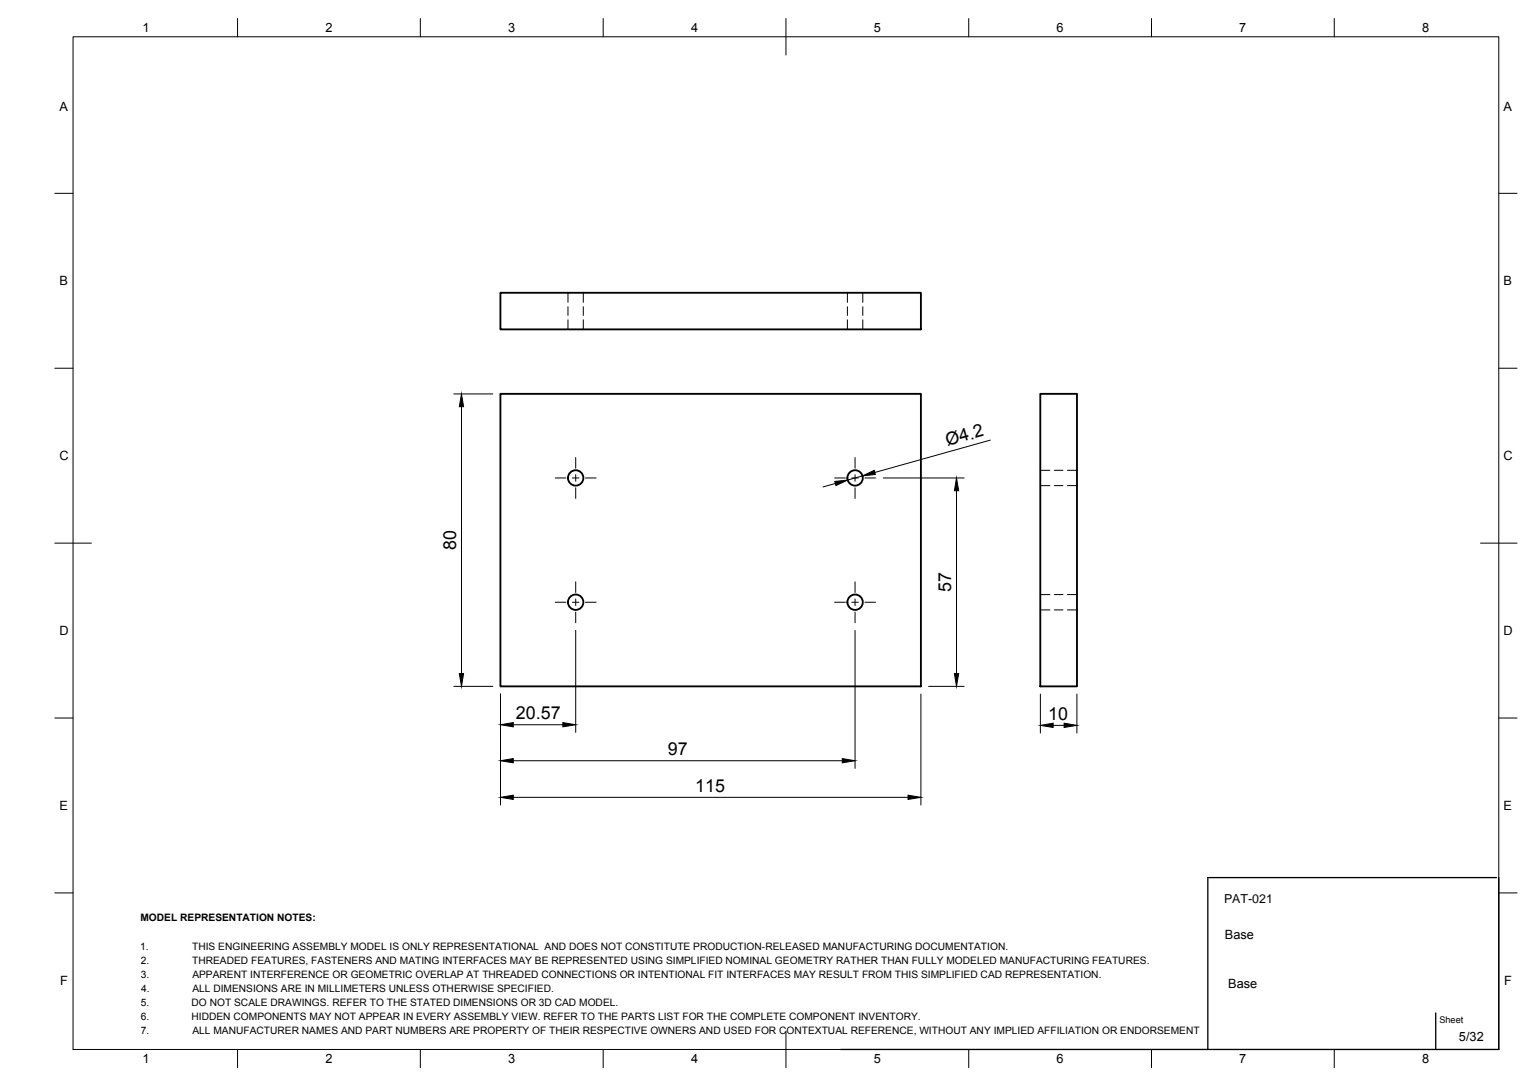
ISO-10303-21;
HEADER;
/* Generated by software containing ST-Developer
 * from STEP Tools, Inc. (www.steptools.com) 
 */

FILE_DESCRIPTION(
/* description */ ('Chain-less indexing wheel (Geneva) drive'),
/* implementation_level */ '2;1');

FILE_NAME(
/* name */ 'Base.step',
/* time_stamp */ '2026-10-28T03:25:22-07:00',
/* author */ (''),
/* organization */ (''),
/* preprocessor_version */ 'ST-DEVELOPER v20.2',
/* originating_system */ 'Autodesk Translation Framework v15.17.0.0',
/* authorisation */ '');

FILE_SCHEMA (('AUTOMOTIVE_DESIGN { 1 0 10303 214 3 1 1 }'));
ENDSEC;

DATA;
#10=MECHANICAL_DESIGN_GEOMETRIC_PRESENTATION_REPRESENTATION('',(#303),#10957);
#253=SHAPE_REPRESENTATION_RELATIONSHIP('SRR','None',#11066,#278);
#278=ADVANCED_BREP_SHAPE_REPRESENTATION('',(#336),#10929);
#303=STYLED_ITEM('',(#11266),#336);
#336=MANIFOLD_SOLID_BREP('Body1',#5699);
#367=FACE_BOUND('',#994,.T.);
#368=FACE_BOUND('',#995,.T.);
#369=FACE_BOUND('',#996,.T.);
#370=FACE_BOUND('',#997,.T.);
#371=FACE_BOUND('',#999,.T.);
#372=FACE_BOUND('',#1000,.T.);
#373=FACE_BOUND('',#1001,.T.);
#374=FACE_BOUND('',#1002,.T.);
#472=PLANE('',#6025);
#473=PLANE('',#6026);
#474=PLANE('',#6027);
#475=PLANE('',#6028);
#476=PLANE('',#6029);
#477=PLANE('',#6030);
#652=FACE_OUTER_BOUND('',#985,.T.);
#653=FACE_OUTER_BOUND('',#986,.T.);
#654=FACE_OUTER_BOUND('',#987,.T.);
#655=FACE_OUTER_BOUND('',#988,.T.);
#656=FACE_OUTER_BOUND('',#989,.T.);
#657=FACE_OUTER_BOUND('',#990,.T.);
#658=FACE_OUTER_BOUND('',#991,.T.);
#659=FACE_OUTER_BOUND('',#992,.T.);
#660=FACE_OUTER_BOUND('',#993,.T.);
#661=FACE_OUTER_BOUND('',#998,.T.);
#985=EDGE_LOOP('',(#3747,#3748,#3749,#3750));
#986=EDGE_LOOP('',(#3751,#3752,#3753,#3754));
#987=EDGE_LOOP('',(#3755,#3756,#3757,#3758));
#988=EDGE_LOOP('',(#3759,#3760,#3761,#3762));
#989=EDGE_LOOP('',(#3763,#3764,#3765,#3766));
#990=EDGE_LOOP('',(#3767,#3768,#3769,#3770));
#991=EDGE_LOOP('',(#3771,#3772,#3773,#3774));
#992=EDGE_LOOP('',(#3775,#3776,#3777,#3778));
#993=EDGE_LOOP('',(#3779,#3780,#3781,#3782));
#994=EDGE_LOOP('',(#3783));
#995=EDGE_LOOP('',(#3784));
#996=EDGE_LOOP('',(#3785));
#997=EDGE_LOOP('',(#3786));
#998=EDGE_LOOP('',(#3787,#3788,#3789,#3790));
#999=EDGE_LOOP('',(#3791));
#1000=EDGE_LOOP('',(#3792));
#1001=EDGE_LOOP('',(#3793));
#1002=EDGE_LOOP('',(#3794));
#1423=LINE('',#8608,#1797);
#1424=LINE('',#8614,#1798);
#1425=LINE('',#8620,#1799);
#1426=LINE('',#8626,#1800);
#1427=LINE('',#8631,#1801);
#1428=LINE('',#8633,#1802);
#1429=LINE('',#8635,#1803);
#1430=LINE('',#8636,#1804);
#1431=LINE('',#8639,#1805);
#1432=LINE('',#8641,#1806);
#1433=LINE('',#8642,#1807);
#1434=LINE('',#8645,#1808);
#1435=LINE('',#8647,#1809);
#1436=LINE('',#8648,#1810);
#1437=LINE('',#8650,#1811);
#1438=LINE('',#8651,#1812);
#1797=VECTOR('',#6759,0.21);
#1798=VECTOR('',#6766,0.21);
#1799=VECTOR('',#6773,0.21);
#1800=VECTOR('',#6780,0.21);
#1801=VECTOR('',#6785,1.);
#1802=VECTOR('',#6786,1.);
#1803=VECTOR('',#6787,1.);
#1804=VECTOR('',#6788,1.);
#1805=VECTOR('',#6791,1.);
#1806=VECTOR('',#6792,1.);
#1807=VECTOR('',#6793,1.);
#1808=VECTOR('',#6796,1.);
#1809=VECTOR('',#6797,1.);
#1810=VECTOR('',#6798,1.);
#1811=VECTOR('',#6801,1.);
#1812=VECTOR('',#6802,1.);
#2171=CIRCLE('',#6014,0.21);
#2172=CIRCLE('',#6015,0.21);
#2173=CIRCLE('',#6017,0.21);
#2174=CIRCLE('',#6018,0.21);
#2175=CIRCLE('',#6020,0.21);
#2176=CIRCLE('',#6021,0.21);
#2177=CIRCLE('',#6023,0.21);
#2178=CIRCLE('',#6024,0.21);
#2505=VERTEX_POINT('',#8605);
#2506=VERTEX_POINT('',#8607);
#2507=VERTEX_POINT('',#8611);
#2508=VERTEX_POINT('',#8613);
#2509=VERTEX_POINT('',#8617);
#2510=VERTEX_POINT('',#8619);
#2511=VERTEX_POINT('',#8623);
#2512=VERTEX_POINT('',#8625);
#2513=VERTEX_POINT('',#8629);
#2514=VERTEX_POINT('',#8630);
#2515=VERTEX_POINT('',#8632);
#2516=VERTEX_POINT('',#8634);
#2517=VERTEX_POINT('',#8638);
#2518=VERTEX_POINT('',#8640);
#2519=VERTEX_POINT('',#8644);
#2520=VERTEX_POINT('',#8646);
#2999=EDGE_CURVE('',#2505,#2505,#2171,.T.);
#3000=EDGE_CURVE('',#2505,#2506,#1423,.T.);
#3001=EDGE_CURVE('',#2506,#2506,#2172,.T.);
#3002=EDGE_CURVE('',#2507,#2507,#2173,.T.);
#3003=EDGE_CURVE('',#2507,#2508,#1424,.T.);
#3004=EDGE_CURVE('',#2508,#2508,#2174,.T.);
#3005=EDGE_CURVE('',#2509,#2509,#2175,.T.);
#3006=EDGE_CURVE('',#2509,#2510,#1425,.T.);
#3007=EDGE_CURVE('',#2510,#2510,#2176,.T.);
#3008=EDGE_CURVE('',#2511,#2511,#2177,.T.);
#3009=EDGE_CURVE('',#2511,#2512,#1426,.T.);
#3010=EDGE_CURVE('',#2512,#2512,#2178,.T.);
#3011=EDGE_CURVE('',#2513,#2514,#1427,.T.);
#3012=EDGE_CURVE('',#2514,#2515,#1428,.T.);
#3013=EDGE_CURVE('',#2516,#2515,#1429,.T.);
#3014=EDGE_CURVE('',#2513,#2516,#1430,.T.);
#3015=EDGE_CURVE('',#2517,#2513,#1431,.T.);
#3016=EDGE_CURVE('',#2518,#2516,#1432,.T.);
#3017=EDGE_CURVE('',#2517,#2518,#1433,.T.);
#3018=EDGE_CURVE('',#2519,#2517,#1434,.T.);
#3019=EDGE_CURVE('',#2520,#2518,#1435,.T.);
#3020=EDGE_CURVE('',#2519,#2520,#1436,.T.);
#3021=EDGE_CURVE('',#2514,#2519,#1437,.T.);
#3022=EDGE_CURVE('',#2515,#2520,#1438,.T.);
#3747=ORIENTED_EDGE('',*,*,#2999,.F.);
#3748=ORIENTED_EDGE('',*,*,#3000,.T.);
#3749=ORIENTED_EDGE('',*,*,#3001,.F.);
#3750=ORIENTED_EDGE('',*,*,#3000,.F.);
#3751=ORIENTED_EDGE('',*,*,#3002,.F.);
#3752=ORIENTED_EDGE('',*,*,#3003,.T.);
#3753=ORIENTED_EDGE('',*,*,#3004,.F.);
#3754=ORIENTED_EDGE('',*,*,#3003,.F.);
#3755=ORIENTED_EDGE('',*,*,#3005,.F.);
#3756=ORIENTED_EDGE('',*,*,#3006,.T.);
#3757=ORIENTED_EDGE('',*,*,#3007,.F.);
#3758=ORIENTED_EDGE('',*,*,#3006,.F.);
#3759=ORIENTED_EDGE('',*,*,#3008,.F.);
#3760=ORIENTED_EDGE('',*,*,#3009,.T.);
#3761=ORIENTED_EDGE('',*,*,#3010,.F.);
#3762=ORIENTED_EDGE('',*,*,#3009,.F.);
#3763=ORIENTED_EDGE('',*,*,#3011,.T.);
#3764=ORIENTED_EDGE('',*,*,#3012,.T.);
#3765=ORIENTED_EDGE('',*,*,#3013,.F.);
#3766=ORIENTED_EDGE('',*,*,#3014,.F.);
#3767=ORIENTED_EDGE('',*,*,#3015,.T.);
#3768=ORIENTED_EDGE('',*,*,#3014,.T.);
#3769=ORIENTED_EDGE('',*,*,#3016,.F.);
#3770=ORIENTED_EDGE('',*,*,#3017,.F.);
#3771=ORIENTED_EDGE('',*,*,#3018,.T.);
#3772=ORIENTED_EDGE('',*,*,#3017,.T.);
#3773=ORIENTED_EDGE('',*,*,#3019,.F.);
#3774=ORIENTED_EDGE('',*,*,#3020,.F.);
#3775=ORIENTED_EDGE('',*,*,#3021,.T.);
#3776=ORIENTED_EDGE('',*,*,#3020,.T.);
#3777=ORIENTED_EDGE('',*,*,#3022,.F.);
#3778=ORIENTED_EDGE('',*,*,#3012,.F.);
#3779=ORIENTED_EDGE('',*,*,#3022,.T.);
#3780=ORIENTED_EDGE('',*,*,#3019,.T.);
#3781=ORIENTED_EDGE('',*,*,#3016,.T.);
#3782=ORIENTED_EDGE('',*,*,#3013,.T.);
#3783=ORIENTED_EDGE('',*,*,#3001,.T.);
#3784=ORIENTED_EDGE('',*,*,#3004,.T.);
#3785=ORIENTED_EDGE('',*,*,#3007,.T.);
#3786=ORIENTED_EDGE('',*,*,#3010,.T.);
#3787=ORIENTED_EDGE('',*,*,#3021,.F.);
#3788=ORIENTED_EDGE('',*,*,#3011,.F.);
#3789=ORIENTED_EDGE('',*,*,#3015,.F.);
#3790=ORIENTED_EDGE('',*,*,#3018,.F.);
#3791=ORIENTED_EDGE('',*,*,#2999,.T.);
#3792=ORIENTED_EDGE('',*,*,#3002,.T.);
#3793=ORIENTED_EDGE('',*,*,#3005,.T.);
#3794=ORIENTED_EDGE('',*,*,#3008,.T.);
#5243=CYLINDRICAL_SURFACE('',#6013,0.21);
#5244=CYLINDRICAL_SURFACE('',#6016,0.21);
#5245=CYLINDRICAL_SURFACE('',#6019,0.21);
#5246=CYLINDRICAL_SURFACE('',#6022,0.21);
#5366=ADVANCED_FACE('',(#652),#5243,.F.);
#5367=ADVANCED_FACE('',(#653),#5244,.F.);
#5368=ADVANCED_FACE('',(#654),#5245,.F.);
#5369=ADVANCED_FACE('',(#655),#5246,.F.);
#5370=ADVANCED_FACE('',(#656),#472,.T.);
#5371=ADVANCED_FACE('',(#657),#473,.T.);
#5372=ADVANCED_FACE('',(#658),#474,.T.);
#5373=ADVANCED_FACE('',(#659),#475,.T.);
#5374=ADVANCED_FACE('',(#660,#367,#368,#369,#370),#476,.T.);
#5375=ADVANCED_FACE('',(#661,#371,#372,#373,#374),#477,.F.);
#5699=CLOSED_SHELL('',(#5366,#5367,#5368,#5369,#5370,#5371,#5372,#5373,
#5374,#5375));
#6012=AXIS2_PLACEMENT_3D('',#8603,#6753,#6754);
#6013=AXIS2_PLACEMENT_3D('',#8604,#6755,#6756);
#6014=AXIS2_PLACEMENT_3D('',#8606,#6757,#6758);
#6015=AXIS2_PLACEMENT_3D('',#8609,#6760,#6761);
#6016=AXIS2_PLACEMENT_3D('',#8610,#6762,#6763);
#6017=AXIS2_PLACEMENT_3D('',#8612,#6764,#6765);
#6018=AXIS2_PLACEMENT_3D('',#8615,#6767,#6768);
#6019=AXIS2_PLACEMENT_3D('',#8616,#6769,#6770);
#6020=AXIS2_PLACEMENT_3D('',#8618,#6771,#6772);
#6021=AXIS2_PLACEMENT_3D('',#8621,#6774,#6775);
#6022=AXIS2_PLACEMENT_3D('',#8622,#6776,#6777);
#6023=AXIS2_PLACEMENT_3D('',#8624,#6778,#6779);
#6024=AXIS2_PLACEMENT_3D('',#8627,#6781,#6782);
#6025=AXIS2_PLACEMENT_3D('',#8628,#6783,#6784);
#6026=AXIS2_PLACEMENT_3D('',#8637,#6789,#6790);
#6027=AXIS2_PLACEMENT_3D('',#8643,#6794,#6795);
#6028=AXIS2_PLACEMENT_3D('',#8649,#6799,#6800);
#6029=AXIS2_PLACEMENT_3D('',#8652,#6803,#6804);
#6030=AXIS2_PLACEMENT_3D('',#8653,#6805,#6806);
#6753=DIRECTION('axis',(0.,0.,1.));
#6754=DIRECTION('refdir',(1.,0.,0.));
#6755=DIRECTION('center_axis',(0.,0.,1.));
#6756=DIRECTION('ref_axis',(1.,0.,0.));
#6757=DIRECTION('center_axis',(0.,0.,1.));
#6758=DIRECTION('ref_axis',(1.,0.,0.));
#6759=DIRECTION('',(0.,0.,1.));
#6760=DIRECTION('center_axis',(0.,0.,-1.));
#6761=DIRECTION('ref_axis',(1.,0.,0.));
#6762=DIRECTION('center_axis',(0.,0.,1.));
#6763=DIRECTION('ref_axis',(1.,0.,0.));
#6764=DIRECTION('center_axis',(0.,0.,1.));
#6765=DIRECTION('ref_axis',(1.,0.,0.));
#6766=DIRECTION('',(0.,0.,1.));
#6767=DIRECTION('center_axis',(0.,0.,-1.));
#6768=DIRECTION('ref_axis',(1.,0.,0.));
#6769=DIRECTION('center_axis',(0.,0.,1.));
#6770=DIRECTION('ref_axis',(1.,0.,0.));
#6771=DIRECTION('center_axis',(0.,0.,1.));
#6772=DIRECTION('ref_axis',(1.,0.,0.));
#6773=DIRECTION('',(0.,0.,1.));
#6774=DIRECTION('center_axis',(0.,0.,-1.));
#6775=DIRECTION('ref_axis',(1.,0.,0.));
#6776=DIRECTION('center_axis',(0.,0.,1.));
#6777=DIRECTION('ref_axis',(1.,0.,0.));
#6778=DIRECTION('center_axis',(0.,0.,1.));
#6779=DIRECTION('ref_axis',(1.,0.,0.));
#6780=DIRECTION('',(0.,0.,1.));
#6781=DIRECTION('center_axis',(0.,0.,-1.));
#6782=DIRECTION('ref_axis',(1.,0.,0.));
#6783=DIRECTION('center_axis',(0.,1.,0.));
#6784=DIRECTION('ref_axis',(-1.,0.,0.));
#6785=DIRECTION('',(-1.,0.,0.));
#6786=DIRECTION('',(0.,0.,1.));
#6787=DIRECTION('',(-1.,0.,0.));
#6788=DIRECTION('',(0.,0.,1.));
#6789=DIRECTION('center_axis',(1.,0.,0.));
#6790=DIRECTION('ref_axis',(0.,1.,0.));
#6791=DIRECTION('',(0.,1.,0.));
#6792=DIRECTION('',(0.,1.,0.));
#6793=DIRECTION('',(0.,0.,1.));
#6794=DIRECTION('center_axis',(0.,-1.,0.));
#6795=DIRECTION('ref_axis',(1.,0.,0.));
#6796=DIRECTION('',(1.,0.,0.));
#6797=DIRECTION('',(1.,0.,0.));
#6798=DIRECTION('',(0.,0.,1.));
#6799=DIRECTION('center_axis',(-1.,0.,0.));
#6800=DIRECTION('ref_axis',(0.,-1.,0.));
#6801=DIRECTION('',(0.,-1.,0.));
#6802=DIRECTION('',(0.,-1.,0.));
#6803=DIRECTION('center_axis',(0.,0.,1.));
#6804=DIRECTION('ref_axis',(1.,0.,0.));
#6805=DIRECTION('center_axis',(0.,0.,1.));
#6806=DIRECTION('ref_axis',(1.,0.,0.));
#8603=CARTESIAN_POINT('',(0.,0.,0.));
#8604=CARTESIAN_POINT('Origin',(5.94264068711928,-1.7,-0.1));
#8605=CARTESIAN_POINT('',(5.73264068711928,-1.7,0.));
#8606=CARTESIAN_POINT('Origin',(5.94264068711928,-1.7,0.));
#8607=CARTESIAN_POINT('',(5.73264068711928,-1.7,1.));
#8608=CARTESIAN_POINT('',(5.73264068711928,-1.7,-0.1));
#8609=CARTESIAN_POINT('Origin',(5.94264068711928,-1.7,1.));
#8610=CARTESIAN_POINT('Origin',(-1.7,1.7,-0.1));
#8611=CARTESIAN_POINT('',(-1.91,1.7,0.));
#8612=CARTESIAN_POINT('Origin',(-1.7,1.7,0.));
#8613=CARTESIAN_POINT('',(-1.91,1.7,1.));
#8614=CARTESIAN_POINT('',(-1.91,1.7,-0.1));
#8615=CARTESIAN_POINT('Origin',(-1.7,1.7,1.));
#8616=CARTESIAN_POINT('Origin',(-1.7,-1.7,-0.1));
#8617=CARTESIAN_POINT('',(-1.91,-1.7,0.));
#8618=CARTESIAN_POINT('Origin',(-1.7,-1.7,0.));
#8619=CARTESIAN_POINT('',(-1.91,-1.7,1.));
#8620=CARTESIAN_POINT('',(-1.91,-1.7,-0.1));
#8621=CARTESIAN_POINT('Origin',(-1.7,-1.7,1.));
#8622=CARTESIAN_POINT('Origin',(5.94264068711928,1.7,-0.1));
#8623=CARTESIAN_POINT('',(5.73264068711928,1.7,0.));
#8624=CARTESIAN_POINT('Origin',(5.94264068711928,1.7,0.));
#8625=CARTESIAN_POINT('',(5.73264068711928,1.7,1.));
#8626=CARTESIAN_POINT('',(5.73264068711928,1.7,-0.1));
#8627=CARTESIAN_POINT('Origin',(5.94264068711928,1.7,1.));
#8628=CARTESIAN_POINT('Origin',(8.,4.,0.));
#8629=CARTESIAN_POINT('',(8.,4.,0.));
#8630=CARTESIAN_POINT('',(-3.5,4.,0.));
#8631=CARTESIAN_POINT('',(8.,4.,0.));
#8632=CARTESIAN_POINT('',(-3.5,4.,1.));
#8633=CARTESIAN_POINT('',(-3.5,4.,0.));
#8634=CARTESIAN_POINT('',(8.,4.,1.));
#8635=CARTESIAN_POINT('',(8.,4.,1.));
#8636=CARTESIAN_POINT('',(8.,4.,0.));
#8637=CARTESIAN_POINT('Origin',(8.,-4.,0.));
#8638=CARTESIAN_POINT('',(8.,-4.,0.));
#8639=CARTESIAN_POINT('',(8.,-4.,0.));
#8640=CARTESIAN_POINT('',(8.,-4.,1.));
#8641=CARTESIAN_POINT('',(8.,-4.,1.));
#8642=CARTESIAN_POINT('',(8.,-4.,0.));
#8643=CARTESIAN_POINT('Origin',(-3.5,-4.,0.));
#8644=CARTESIAN_POINT('',(-3.5,-4.,0.));
#8645=CARTESIAN_POINT('',(-3.5,-4.,0.));
#8646=CARTESIAN_POINT('',(-3.5,-4.,1.));
#8647=CARTESIAN_POINT('',(-3.5,-4.,1.));
#8648=CARTESIAN_POINT('',(-3.5,-4.,0.));
#8649=CARTESIAN_POINT('Origin',(-3.5,4.,0.));
#8650=CARTESIAN_POINT('',(-3.5,4.,0.));
#8651=CARTESIAN_POINT('',(-3.5,4.,1.));
#8652=CARTESIAN_POINT('Origin',(2.25,0.,1.));
#8653=CARTESIAN_POINT('Origin',(2.25,0.,0.));
#10898=UNCERTAINTY_MEASURE_WITH_UNIT(LENGTH_MEASURE(0.001),#10958,
'DISTANCE_ACCURACY_VALUE',
'Maximum model space distance between geometric entities at asserted c
onnectivities');
#10926=UNCERTAINTY_MEASURE_WITH_UNIT(LENGTH_MEASURE(0.001),#10958,
'DISTANCE_ACCURACY_VALUE',
'Maximum model space distance between geometric entities at asserted c
onnectivities');
#10929=(
GEOMETRIC_REPRESENTATION_CONTEXT(3)
GLOBAL_UNCERTAINTY_ASSIGNED_CONTEXT((#10898))
GLOBAL_UNIT_ASSIGNED_CONTEXT((#10958,#10960,#10961))
REPRESENTATION_CONTEXT('','3D')
);
#10957=(
GEOMETRIC_REPRESENTATION_CONTEXT(3)
GLOBAL_UNCERTAINTY_ASSIGNED_CONTEXT((#10926))
GLOBAL_UNIT_ASSIGNED_CONTEXT((#10958,#10960,#10961))
REPRESENTATION_CONTEXT('','3D')
);
#10958=(
LENGTH_UNIT()
NAMED_UNIT(*)
SI_UNIT(.CENTI.,.METRE.)
);
#10960=(
NAMED_UNIT(*)
PLANE_ANGLE_UNIT()
SI_UNIT($,.RADIAN.)
);
#10961=(
NAMED_UNIT(*)
SI_UNIT($,.STERADIAN.)
SOLID_ANGLE_UNIT()
);
#10964=SHAPE_DEFINITION_REPRESENTATION(#10994,#11066);
#10994=PRODUCT_DEFINITION_SHAPE('',$,#11097);
#11066=SHAPE_REPRESENTATION('',(#6012),#10929);
#11094=PRODUCT_DEFINITION_CONTEXT('part definition',#11186,'design');
#11097=PRODUCT_DEFINITION('Base','Base',#11127,#11094);
#11127=PRODUCT_DEFINITION_FORMATION('',$,#11190);
#11186=APPLICATION_CONTEXT(
'Core Data for Automotive Mechanical Design Process');
#11187=PRODUCT_CONTEXT('part definition',#11186,'mechanical');
#11190=PRODUCT('Base','Base','Base',(#11187));
#11260=COLOUR_RGB('Dark Blue',0.08,0.2,0.34);
#11261=FILL_AREA_STYLE_COLOUR('',#11260);
#11262=FILL_AREA_STYLE('',(#11261));
#11263=SURFACE_STYLE_FILL_AREA(#11262);
#11264=SURFACE_SIDE_STYLE('',(#11263));
#11265=SURFACE_STYLE_USAGE(.BOTH.,#11264);
#11266=PRESENTATION_STYLE_ASSIGNMENT((#11265));
ENDSEC;
END-ISO-10303-21;
